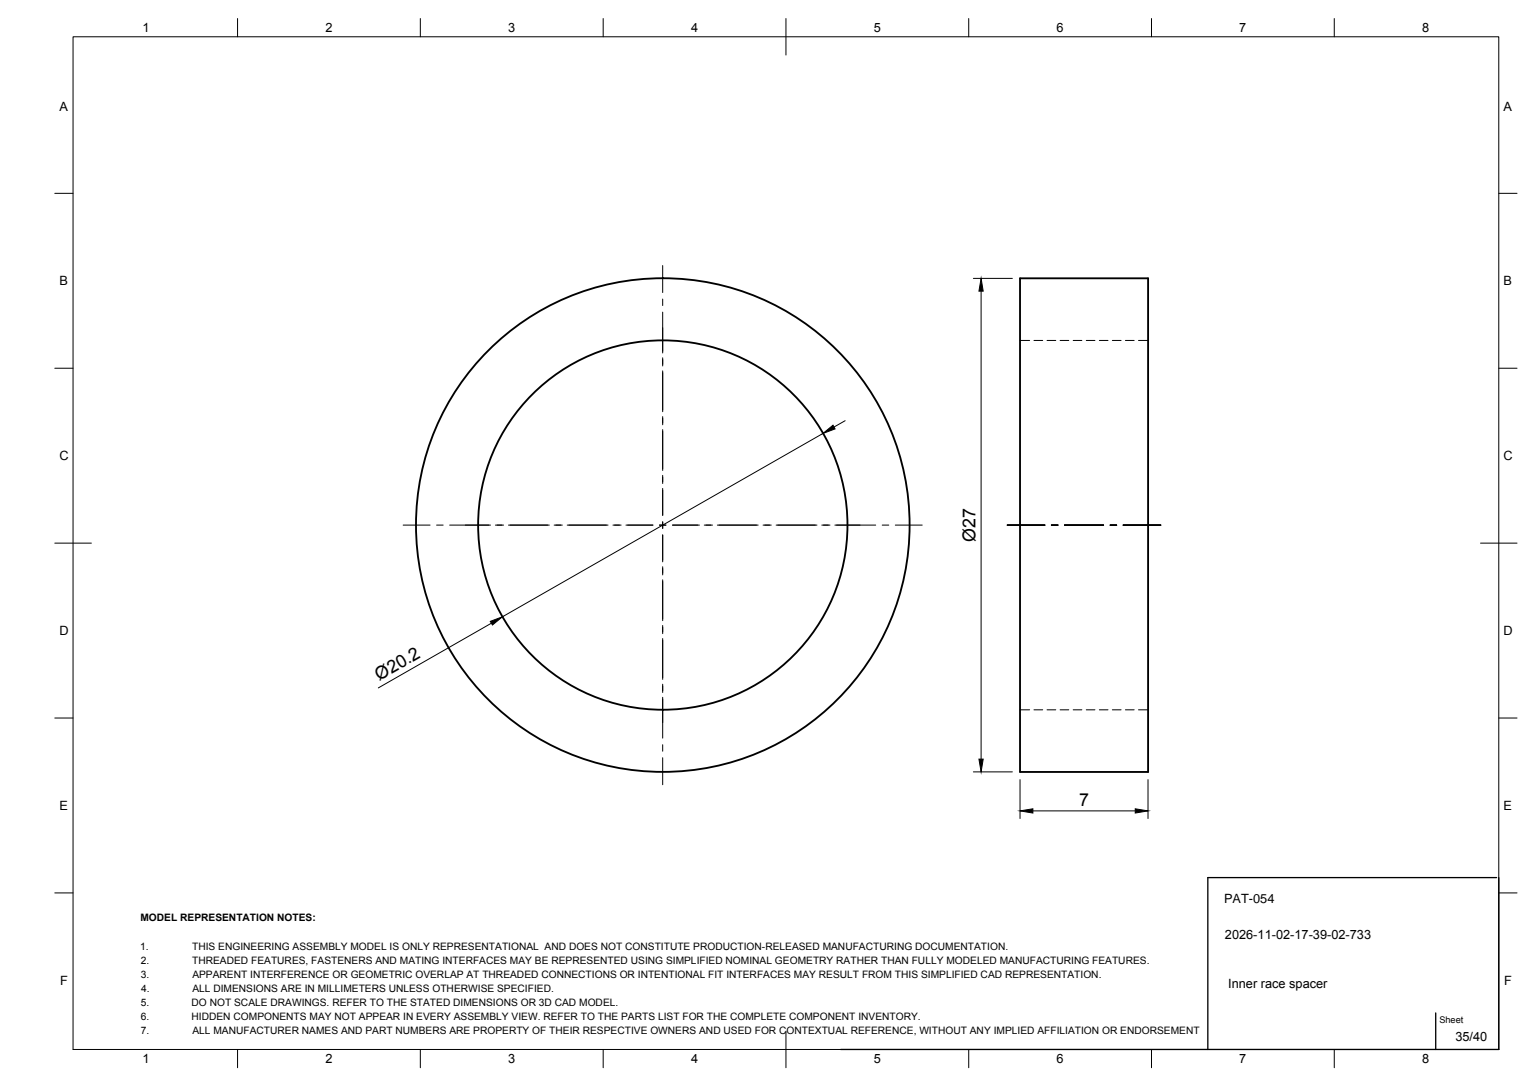
ISO-10303-21;
HEADER;
/* Generated by software containing ST-Developer
 * from STEP Tools, Inc. (www.steptools.com) 
 */

FILE_DESCRIPTION(
/* description */ ('PAT-054'),
/* implementation_level */ '2;1');

FILE_NAME(
/* name */ 'Inner race spacer.step',
/* time_stamp */ '2026-10-29T16:38:13-07:00',
/* author */ (''),
/* organization */ (''),
/* preprocessor_version */ 'ST-DEVELOPER v20.2',
/* originating_system */ 'Autodesk Translation Framework v15.17.0.0',
/* authorisation */ '');

FILE_SCHEMA (('AUTOMOTIVE_DESIGN { 1 0 10303 214 3 1 1 }'));
ENDSEC;

DATA;
#10=MECHANICAL_DESIGN_GEOMETRIC_PRESENTATION_REPRESENTATION('',(#949),#33981);
#846=SHAPE_REPRESENTATION_RELATIONSHIP('SRR','None',#34224,#890);
#890=ADVANCED_BREP_SHAPE_REPRESENTATION('',(#1004),#33972);
#949=STYLED_ITEM('',(#34517),#1004);
#1004=MANIFOLD_SOLID_BREP('Body1',#13064);
#1208=FACE_BOUND('',#3145,.T.);
#1209=FACE_BOUND('',#3147,.T.);
#1525=PLANE('',#14708);
#1526=PLANE('',#14709);
#2223=FACE_OUTER_BOUND('',#3142,.T.);
#2224=FACE_OUTER_BOUND('',#3143,.T.);
#2225=FACE_OUTER_BOUND('',#3144,.T.);
#2226=FACE_OUTER_BOUND('',#3146,.T.);
#3142=EDGE_LOOP('',(#11669,#11670,#11671,#11672));
#3143=EDGE_LOOP('',(#11673,#11674,#11675,#11676));
#3144=EDGE_LOOP('',(#11677));
#3145=EDGE_LOOP('',(#11678));
#3146=EDGE_LOOP('',(#11679));
#3147=EDGE_LOOP('',(#11680));
#4070=LINE('',#33367,#5004);
#4071=LINE('',#33373,#5005);
#5004=VECTOR('',#18013,1.01);
#5005=VECTOR('',#18020,1.35);
#5526=CIRCLE('',#14703,1.01);
#5527=CIRCLE('',#14704,1.01);
#5528=CIRCLE('',#14706,1.35);
#5529=CIRCLE('',#14707,1.35);
#6642=VERTEX_POINT('',#33364);
#6643=VERTEX_POINT('',#33366);
#6644=VERTEX_POINT('',#33370);
#6645=VERTEX_POINT('',#33372);
#8334=EDGE_CURVE('',#6642,#6642,#5526,.T.);
#8335=EDGE_CURVE('',#6642,#6643,#4070,.T.);
#8336=EDGE_CURVE('',#6643,#6643,#5527,.T.);
#8337=EDGE_CURVE('',#6644,#6644,#5528,.T.);
#8338=EDGE_CURVE('',#6644,#6645,#4071,.T.);
#8339=EDGE_CURVE('',#6645,#6645,#5529,.T.);
#11669=ORIENTED_EDGE('',*,*,#8334,.F.);
#11670=ORIENTED_EDGE('',*,*,#8335,.T.);
#11671=ORIENTED_EDGE('',*,*,#8336,.T.);
#11672=ORIENTED_EDGE('',*,*,#8335,.F.);
#11673=ORIENTED_EDGE('',*,*,#8337,.F.);
#11674=ORIENTED_EDGE('',*,*,#8338,.T.);
#11675=ORIENTED_EDGE('',*,*,#8339,.T.);
#11676=ORIENTED_EDGE('',*,*,#8338,.F.);
#11677=ORIENTED_EDGE('',*,*,#8337,.T.);
#11678=ORIENTED_EDGE('',*,*,#8334,.T.);
#11679=ORIENTED_EDGE('',*,*,#8339,.F.);
#11680=ORIENTED_EDGE('',*,*,#8336,.F.);
#12268=CYLINDRICAL_SURFACE('',#14702,1.01);
#12269=CYLINDRICAL_SURFACE('',#14705,1.35);
#12935=ADVANCED_FACE('',(#2223),#12268,.F.);
#12936=ADVANCED_FACE('',(#2224),#12269,.T.);
#12937=ADVANCED_FACE('',(#2225,#1208),#1525,.T.);
#12938=ADVANCED_FACE('',(#2226,#1209),#1526,.F.);
#13064=CLOSED_SHELL('',(#12935,#12936,#12937,#12938));
#14701=AXIS2_PLACEMENT_3D('',#33362,#18007,#18008);
#14702=AXIS2_PLACEMENT_3D('',#33363,#18009,#18010);
#14703=AXIS2_PLACEMENT_3D('',#33365,#18011,#18012);
#14704=AXIS2_PLACEMENT_3D('',#33368,#18014,#18015);
#14705=AXIS2_PLACEMENT_3D('',#33369,#18016,#18017);
#14706=AXIS2_PLACEMENT_3D('',#33371,#18018,#18019);
#14707=AXIS2_PLACEMENT_3D('',#33374,#18021,#18022);
#14708=AXIS2_PLACEMENT_3D('',#33375,#18023,#18024);
#14709=AXIS2_PLACEMENT_3D('',#33376,#18025,#18026);
#18007=DIRECTION('axis',(0.,0.,1.));
#18008=DIRECTION('refdir',(1.,0.,0.));
#18009=DIRECTION('center_axis',(1.,0.,0.));
#18010=DIRECTION('ref_axis',(0.,0.,-1.));
#18011=DIRECTION('center_axis',(-1.,0.,0.));
#18012=DIRECTION('ref_axis',(0.,0.,-1.));
#18013=DIRECTION('',(-1.,0.,0.));
#18014=DIRECTION('center_axis',(-1.,0.,0.));
#18015=DIRECTION('ref_axis',(0.,0.,-1.));
#18016=DIRECTION('center_axis',(1.,0.,0.));
#18017=DIRECTION('ref_axis',(0.,0.,-1.));
#18018=DIRECTION('center_axis',(1.,0.,0.));
#18019=DIRECTION('ref_axis',(0.,0.,-1.));
#18020=DIRECTION('',(-1.,0.,0.));
#18021=DIRECTION('center_axis',(1.,0.,0.));
#18022=DIRECTION('ref_axis',(0.,0.,-1.));
#18023=DIRECTION('center_axis',(1.,0.,0.));
#18024=DIRECTION('ref_axis',(0.,0.,-1.));
#18025=DIRECTION('center_axis',(1.,0.,0.));
#18026=DIRECTION('ref_axis',(0.,0.,-1.));
#33362=CARTESIAN_POINT('',(0.,0.,0.));
#33363=CARTESIAN_POINT('Origin',(24.7,0.,4.));
#33364=CARTESIAN_POINT('',(25.4,-1.23689326713883E-16,5.01));
#33365=CARTESIAN_POINT('Origin',(25.4,0.,4.));
#33366=CARTESIAN_POINT('',(24.7,-1.23689326713883E-16,5.01));
#33367=CARTESIAN_POINT('',(24.7,-1.23689326713883E-16,5.01));
#33368=CARTESIAN_POINT('Origin',(24.7,0.,4.));
#33369=CARTESIAN_POINT('Origin',(24.7,0.,4.));
#33370=CARTESIAN_POINT('',(25.4,-1.65327317884893E-16,5.35));
#33371=CARTESIAN_POINT('Origin',(25.4,0.,4.));
#33372=CARTESIAN_POINT('',(24.7,-1.65327317884893E-16,5.35));
#33373=CARTESIAN_POINT('',(24.7,-1.65327317884893E-16,5.35));
#33374=CARTESIAN_POINT('Origin',(24.7,0.,4.));
#33375=CARTESIAN_POINT('Origin',(25.4,0.,4.));
#33376=CARTESIAN_POINT('Origin',(24.7,0.,4.));
#33920=UNCERTAINTY_MEASURE_WITH_UNIT(LENGTH_MEASURE(0.001),#33982,
'DISTANCE_ACCURACY_VALUE',
'Maximum model space distance between geometric entities at asserted c
onnectivities');
#33929=UNCERTAINTY_MEASURE_WITH_UNIT(LENGTH_MEASURE(0.001),#33982,
'DISTANCE_ACCURACY_VALUE',
'Maximum model space distance between geometric entities at asserted c
onnectivities');
#33972=(
GEOMETRIC_REPRESENTATION_CONTEXT(3)
GLOBAL_UNCERTAINTY_ASSIGNED_CONTEXT((#33920))
GLOBAL_UNIT_ASSIGNED_CONTEXT((#33982,#33984,#33985))
REPRESENTATION_CONTEXT('','3D')
);
#33981=(
GEOMETRIC_REPRESENTATION_CONTEXT(3)
GLOBAL_UNCERTAINTY_ASSIGNED_CONTEXT((#33929))
GLOBAL_UNIT_ASSIGNED_CONTEXT((#33982,#33984,#33985))
REPRESENTATION_CONTEXT('','3D')
);
#33982=(
LENGTH_UNIT()
NAMED_UNIT(*)
SI_UNIT(.CENTI.,.METRE.)
);
#33984=(
NAMED_UNIT(*)
PLANE_ANGLE_UNIT()
SI_UNIT($,.RADIAN.)
);
#33985=(
NAMED_UNIT(*)
SI_UNIT($,.STERADIAN.)
SOLID_ANGLE_UNIT()
);
#34028=SHAPE_DEFINITION_REPRESENTATION(#34112,#34224);
#34112=PRODUCT_DEFINITION_SHAPE('',$,#34276);
#34224=SHAPE_REPRESENTATION('',(#14701),#33972);
#34233=PRODUCT_DEFINITION_CONTEXT('part definition',#34388,'design');
#34276=PRODUCT_DEFINITION('Inner race spacer','Inner race spacer',#34327,
#34233);
#34327=PRODUCT_DEFINITION_FORMATION('',$,#34432);
#34388=APPLICATION_CONTEXT(
'Core Data for Automotive Mechanical Design Process');
#34389=PRODUCT_CONTEXT('part definition',#34388,'mechanical');
#34432=PRODUCT('Inner race spacer','Inner race spacer',
'Inner race spacer',(#34389));
#34511=COLOUR_RGB('Grey',0.48,0.52,0.57);
#34512=FILL_AREA_STYLE_COLOUR('',#34511);
#34513=FILL_AREA_STYLE('',(#34512));
#34514=SURFACE_STYLE_FILL_AREA(#34513);
#34515=SURFACE_SIDE_STYLE('',(#34514));
#34516=SURFACE_STYLE_USAGE(.BOTH.,#34515);
#34517=PRESENTATION_STYLE_ASSIGNMENT((#34516));
ENDSEC;
END-ISO-10303-21;
